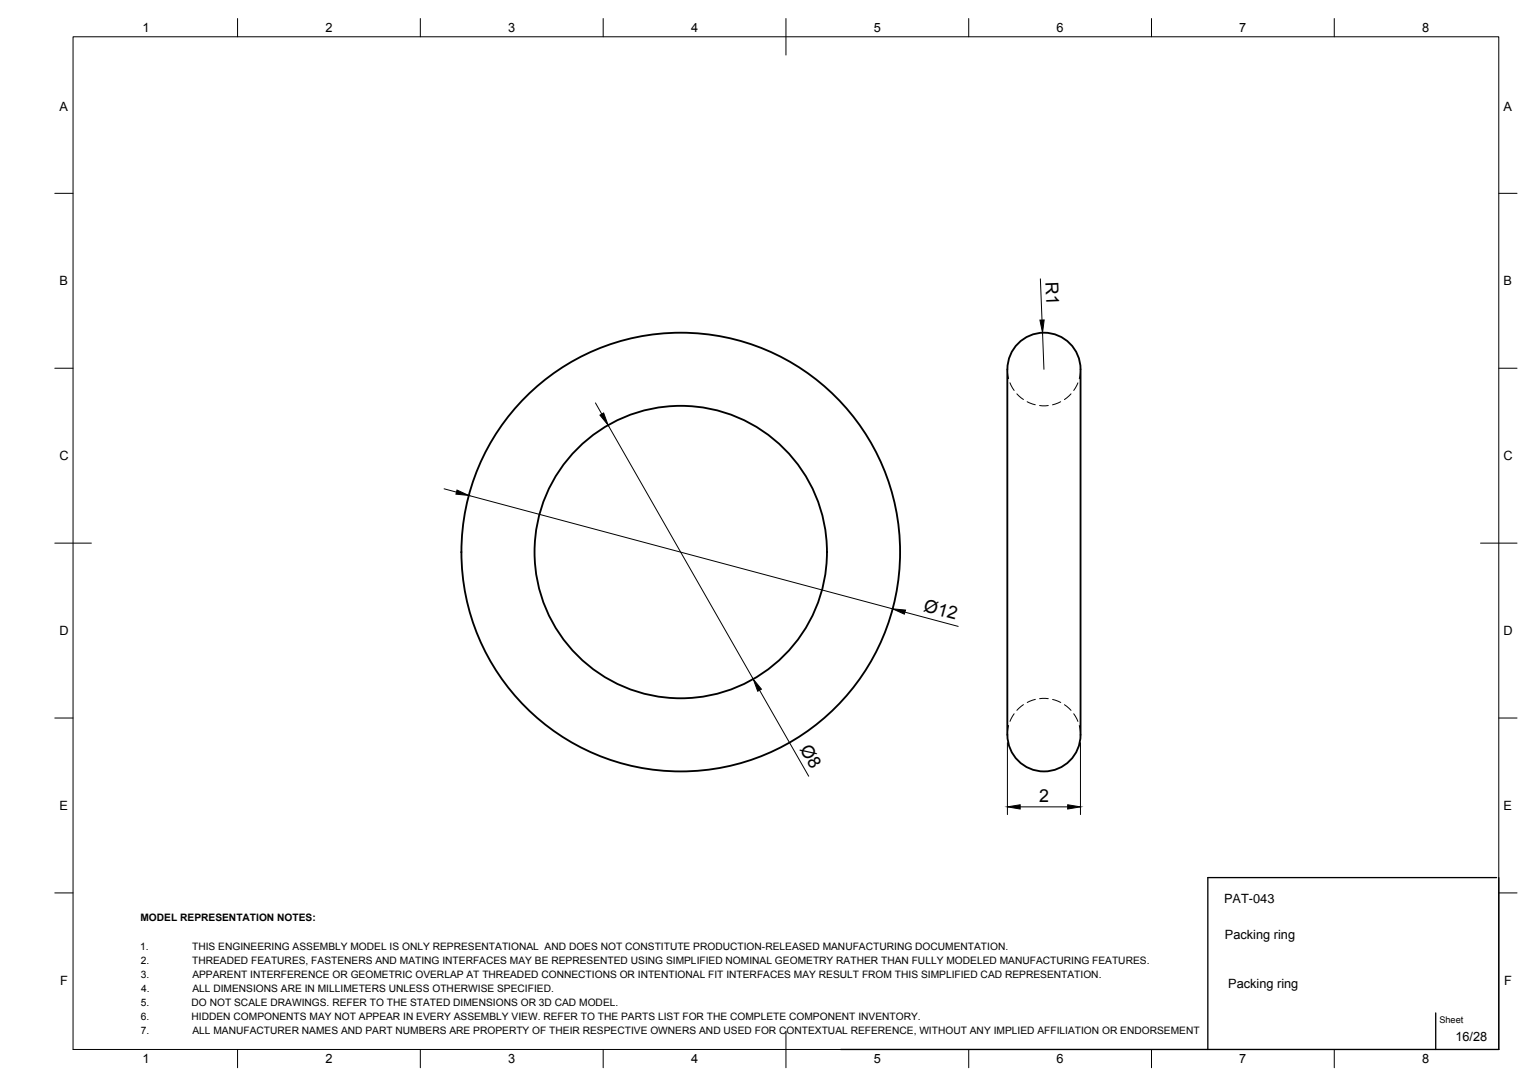
ISO-10303-21;
HEADER;
/* Generated by software containing ST-Developer
 * from STEP Tools, Inc. (www.steptools.com) 
 */

FILE_DESCRIPTION(
/* description */ ('Four-valve pipe header'),
/* implementation_level */ '2;1');

FILE_NAME(
/* name */ 'Packing ring.step',
/* time_stamp */ '2026-10-29T16:56:19-07:00',
/* author */ (''),
/* organization */ (''),
/* preprocessor_version */ 'ST-DEVELOPER v20.2',
/* originating_system */ 'Autodesk Translation Framework v15.17.0.0',
/* authorisation */ '');

FILE_SCHEMA (('AUTOMOTIVE_DESIGN { 1 0 10303 214 3 1 1 }'));
ENDSEC;

DATA;
#10=MECHANICAL_DESIGN_GEOMETRIC_PRESENTATION_REPRESENTATION('',(#342),#10119);
#241=TOROIDAL_SURFACE('',#6233,0.5,0.1);
#290=SHAPE_REPRESENTATION_RELATIONSHIP('SRR','None',#10252,#316);
#316=ADVANCED_BREP_SHAPE_REPRESENTATION('',(#368),#10101);
#342=STYLED_ITEM('',(#10463),#368);
#368=MANIFOLD_SOLID_BREP('Body1',#5588);
#914=FACE_OUTER_BOUND('',#1315,.T.);
#1315=EDGE_LOOP('',(#4501,#4502,#4503,#4504));
#2482=CIRCLE('',#6234,0.1);
#2483=CIRCLE('',#6235,0.4);
#2828=VERTEX_POINT('',#9264);
#3417=EDGE_CURVE('',#2828,#2828,#2482,.T.);
#3418=EDGE_CURVE('',#2828,#2828,#2483,.T.);
#4501=ORIENTED_EDGE('',*,*,#3417,.F.);
#4502=ORIENTED_EDGE('',*,*,#3418,.T.);
#4503=ORIENTED_EDGE('',*,*,#3417,.T.);
#4504=ORIENTED_EDGE('',*,*,#3418,.F.);
#5414=ADVANCED_FACE('',(#914),#241,.T.);
#5588=CLOSED_SHELL('',(#5414));
#6232=AXIS2_PLACEMENT_3D('',#9262,#7447,#7448);
#6233=AXIS2_PLACEMENT_3D('',#9263,#7449,#7450);
#6234=AXIS2_PLACEMENT_3D('',#9265,#7451,#7452);
#6235=AXIS2_PLACEMENT_3D('',#9266,#7453,#7454);
#7447=DIRECTION('axis',(0.,0.,1.));
#7448=DIRECTION('refdir',(1.,0.,0.));
#7449=DIRECTION('center_axis',(0.,0.,1.));
#7450=DIRECTION('ref_axis',(1.,0.,0.));
#7451=DIRECTION('center_axis',(1.22464679914735E-16,-1.,0.));
#7452=DIRECTION('ref_axis',(-1.,-1.22464679914735E-16,0.));
#7453=DIRECTION('center_axis',(0.,0.,-1.));
#7454=DIRECTION('ref_axis',(1.,0.,0.));
#9262=CARTESIAN_POINT('',(0.,0.,0.));
#9263=CARTESIAN_POINT('Origin',(0.,0.,8.1));
#9264=CARTESIAN_POINT('',(-0.4,-4.89858719658941E-17,8.1));
#9265=CARTESIAN_POINT('Origin',(-0.5,-6.12323399573677E-17,8.1));
#9266=CARTESIAN_POINT('Origin',(0.,0.,8.1));
#10070=UNCERTAINTY_MEASURE_WITH_UNIT(LENGTH_MEASURE(0.001),#10120,
'DISTANCE_ACCURACY_VALUE',
'Maximum model space distance between geometric entities at asserted c
onnectivities');
#10088=UNCERTAINTY_MEASURE_WITH_UNIT(LENGTH_MEASURE(0.001),#10120,
'DISTANCE_ACCURACY_VALUE',
'Maximum model space distance between geometric entities at asserted c
onnectivities');
#10101=(
GEOMETRIC_REPRESENTATION_CONTEXT(3)
GLOBAL_UNCERTAINTY_ASSIGNED_CONTEXT((#10070))
GLOBAL_UNIT_ASSIGNED_CONTEXT((#10120,#10122,#10123))
REPRESENTATION_CONTEXT('','3D')
);
#10119=(
GEOMETRIC_REPRESENTATION_CONTEXT(3)
GLOBAL_UNCERTAINTY_ASSIGNED_CONTEXT((#10088))
GLOBAL_UNIT_ASSIGNED_CONTEXT((#10120,#10122,#10123))
REPRESENTATION_CONTEXT('','3D')
);
#10120=(
LENGTH_UNIT()
NAMED_UNIT(*)
SI_UNIT(.CENTI.,.METRE.)
);
#10122=(
NAMED_UNIT(*)
PLANE_ANGLE_UNIT()
SI_UNIT($,.RADIAN.)
);
#10123=(
NAMED_UNIT(*)
SI_UNIT($,.STERADIAN.)
SOLID_ANGLE_UNIT()
);
#10136=SHAPE_DEFINITION_REPRESENTATION(#10166,#10252);
#10166=PRODUCT_DEFINITION_SHAPE('',$,#10283);
#10252=SHAPE_REPRESENTATION('',(#6232),#10101);
#10270=PRODUCT_DEFINITION_CONTEXT('part definition',#10362,'design');
#10283=PRODUCT_DEFINITION('Packing ring','Packing ring',#10313,#10270);
#10313=PRODUCT_DEFINITION_FORMATION('',$,#10376);
#10362=APPLICATION_CONTEXT(
'Core Data for Automotive Mechanical Design Process');
#10363=PRODUCT_CONTEXT('part definition',#10362,'mechanical');
#10376=PRODUCT('Packing ring','Packing ring','Packing ring',(#10363));
#10457=COLOUR_RGB('Sky Blue',0.24,0.69,0.87);
#10458=FILL_AREA_STYLE_COLOUR('',#10457);
#10459=FILL_AREA_STYLE('',(#10458));
#10460=SURFACE_STYLE_FILL_AREA(#10459);
#10461=SURFACE_SIDE_STYLE('',(#10460));
#10462=SURFACE_STYLE_USAGE(.BOTH.,#10461);
#10463=PRESENTATION_STYLE_ASSIGNMENT((#10462));
ENDSEC;
END-ISO-10303-21;
